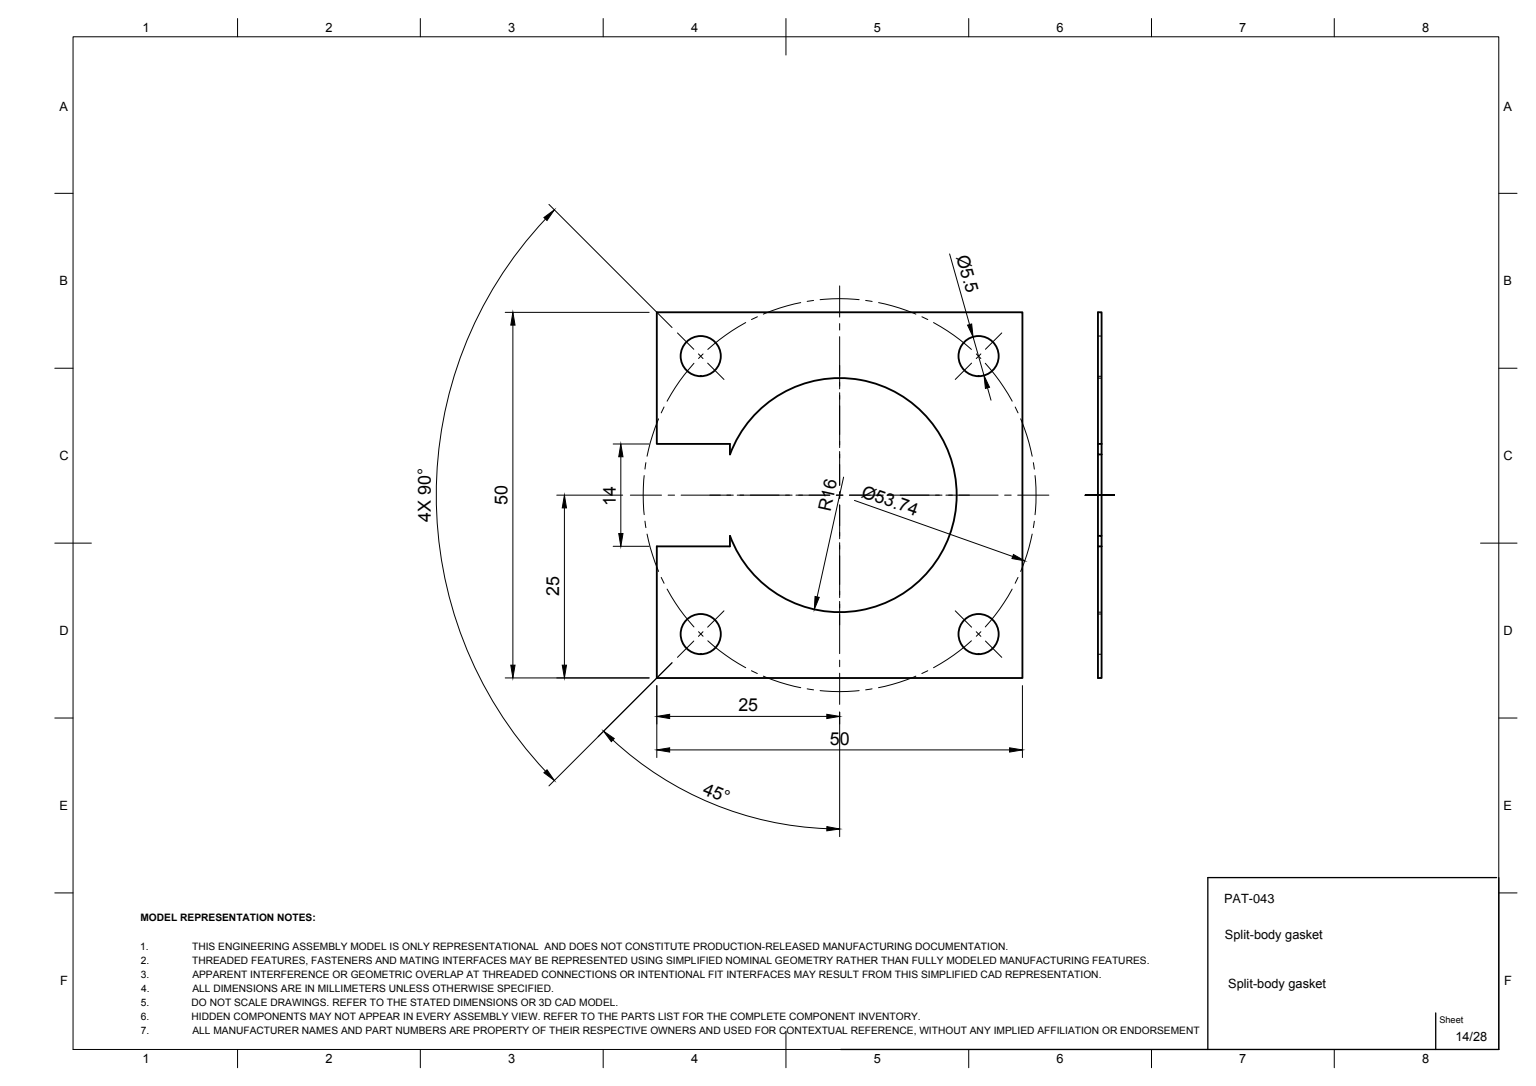
ISO-10303-21;
HEADER;
/* Generated by software containing ST-Developer
 * from STEP Tools, Inc. (www.steptools.com) 
 */

FILE_DESCRIPTION(
/* description */ ('Four-valve pipe header'),
/* implementation_level */ '2;1');

FILE_NAME(
/* name */ 'Split-body gasket.step',
/* time_stamp */ '2026-10-29T16:56:19-07:00',
/* author */ (''),
/* organization */ (''),
/* preprocessor_version */ 'ST-DEVELOPER v20.2',
/* originating_system */ 'Autodesk Translation Framework v15.17.0.0',
/* authorisation */ '');

FILE_SCHEMA (('AUTOMOTIVE_DESIGN { 1 0 10303 214 3 1 1 }'));
ENDSEC;

DATA;
#10=MECHANICAL_DESIGN_GEOMETRIC_PRESENTATION_REPRESENTATION('',(#340),#10119);
#288=SHAPE_REPRESENTATION_RELATIONSHIP('SRR','None',#10250,#314);
#314=ADVANCED_BREP_SHAPE_REPRESENTATION('',(#366),#10099);
#340=STYLED_ITEM('',(#10449),#366);
#366=MANIFOLD_SOLID_BREP('Body1',#5586);
#484=FACE_BOUND('',#1291,.T.);
#485=FACE_BOUND('',#1292,.T.);
#486=FACE_BOUND('',#1293,.T.);
#487=FACE_BOUND('',#1294,.T.);
#488=FACE_BOUND('',#1302,.T.);
#489=FACE_BOUND('',#1303,.T.);
#490=FACE_BOUND('',#1304,.T.);
#491=FACE_BOUND('',#1305,.T.);
#619=PLANE('',#6205);
#620=PLANE('',#6206);
#621=PLANE('',#6207);
#622=PLANE('',#6208);
#623=PLANE('',#6209);
#624=PLANE('',#6211);
#625=PLANE('',#6212);
#626=PLANE('',#6215);
#627=PLANE('',#6216);
#628=PLANE('',#6217);
#629=PLANE('',#6218);
#892=FACE_OUTER_BOUND('',#1282,.T.);
#893=FACE_OUTER_BOUND('',#1283,.T.);
#894=FACE_OUTER_BOUND('',#1284,.T.);
#895=FACE_OUTER_BOUND('',#1285,.T.);
#896=FACE_OUTER_BOUND('',#1286,.T.);
#897=FACE_OUTER_BOUND('',#1287,.T.);
#898=FACE_OUTER_BOUND('',#1288,.T.);
#899=FACE_OUTER_BOUND('',#1289,.T.);
#900=FACE_OUTER_BOUND('',#1290,.T.);
#901=FACE_OUTER_BOUND('',#1295,.T.);
#902=FACE_OUTER_BOUND('',#1296,.T.);
#903=FACE_OUTER_BOUND('',#1297,.T.);
#904=FACE_OUTER_BOUND('',#1298,.T.);
#905=FACE_OUTER_BOUND('',#1299,.T.);
#906=FACE_OUTER_BOUND('',#1300,.T.);
#907=FACE_OUTER_BOUND('',#1301,.T.);
#1282=EDGE_LOOP('',(#4399,#4400,#4401,#4402));
#1283=EDGE_LOOP('',(#4403,#4404,#4405,#4406));
#1284=EDGE_LOOP('',(#4407,#4408,#4409,#4410));
#1285=EDGE_LOOP('',(#4411,#4412,#4413,#4414));
#1286=EDGE_LOOP('',(#4415,#4416,#4417,#4418));
#1287=EDGE_LOOP('',(#4419,#4420,#4421,#4422));
#1288=EDGE_LOOP('',(#4423,#4424,#4425,#4426));
#1289=EDGE_LOOP('',(#4427,#4428,#4429,#4430));
#1290=EDGE_LOOP('',(#4431,#4432,#4433,#4434,#4435,#4436,#4437,#4438,#4439,
#4440));
#1291=EDGE_LOOP('',(#4441));
#1292=EDGE_LOOP('',(#4442));
#1293=EDGE_LOOP('',(#4443));
#1294=EDGE_LOOP('',(#4444));
#1295=EDGE_LOOP('',(#4445,#4446,#4447,#4448));
#1296=EDGE_LOOP('',(#4449,#4450,#4451,#4452));
#1297=EDGE_LOOP('',(#4453,#4454,#4455,#4456));
#1298=EDGE_LOOP('',(#4457,#4458,#4459,#4460));
#1299=EDGE_LOOP('',(#4461,#4462,#4463,#4464));
#1300=EDGE_LOOP('',(#4465,#4466,#4467,#4468));
#1301=EDGE_LOOP('',(#4469,#4470,#4471,#4472,#4473,#4474,#4475,#4476,#4477,
#4478));
#1302=EDGE_LOOP('',(#4479));
#1303=EDGE_LOOP('',(#4480));
#1304=EDGE_LOOP('',(#4481));
#1305=EDGE_LOOP('',(#4482));
#1689=LINE('',#9158,#2107);
#1690=LINE('',#9164,#2108);
#1691=LINE('',#9170,#2109);
#1692=LINE('',#9176,#2110);
#1693=LINE('',#9181,#2111);
#1694=LINE('',#9183,#2112);
#1695=LINE('',#9185,#2113);
#1696=LINE('',#9186,#2114);
#1697=LINE('',#9190,#2115);
#1698=LINE('',#9192,#2116);
#1699=LINE('',#9194,#2117);
#1700=LINE('',#9195,#2118);
#1701=LINE('',#9198,#2119);
#1702=LINE('',#9200,#2120);
#1703=LINE('',#9201,#2121);
#1704=LINE('',#9204,#2122);
#1705=LINE('',#9206,#2123);
#1706=LINE('',#9207,#2124);
#1707=LINE('',#9211,#2125);
#1708=LINE('',#9213,#2126);
#1709=LINE('',#9215,#2127);
#1710=LINE('',#9217,#2128);
#1711=LINE('',#9218,#2129);
#1712=LINE('',#9221,#2130);
#1713=LINE('',#9222,#2131);
#1714=LINE('',#9225,#2132);
#1715=LINE('',#9226,#2133);
#1716=LINE('',#9231,#2134);
#1717=LINE('',#9232,#2135);
#1718=LINE('',#9235,#2136);
#1719=LINE('',#9236,#2137);
#1720=LINE('',#9238,#2138);
#2107=VECTOR('',#7338,0.275);
#2108=VECTOR('',#7345,0.275);
#2109=VECTOR('',#7352,0.275);
#2110=VECTOR('',#7359,0.275);
#2111=VECTOR('',#7364,1.);
#2112=VECTOR('',#7365,1.);
#2113=VECTOR('',#7366,1.);
#2114=VECTOR('',#7367,1.);
#2115=VECTOR('',#7370,1.);
#2116=VECTOR('',#7371,1.);
#2117=VECTOR('',#7372,1.);
#2118=VECTOR('',#7373,1.);
#2119=VECTOR('',#7376,1.);
#2120=VECTOR('',#7377,1.);
#2121=VECTOR('',#7378,1.);
#2122=VECTOR('',#7381,1.);
#2123=VECTOR('',#7382,1.);
#2124=VECTOR('',#7383,1.);
#2125=VECTOR('',#7388,1.);
#2126=VECTOR('',#7389,1.);
#2127=VECTOR('',#7390,1.);
#2128=VECTOR('',#7391,1.);
#2129=VECTOR('',#7392,1.);
#2130=VECTOR('',#7395,1.);
#2131=VECTOR('',#7396,1.);
#2132=VECTOR('',#7399,1.);
#2133=VECTOR('',#7400,1.);
#2134=VECTOR('',#7407,1.);
#2135=VECTOR('',#7408,1.);
#2136=VECTOR('',#7411,1.);
#2137=VECTOR('',#7412,1.);
#2138=VECTOR('',#7415,1.);
#2466=CIRCLE('',#6194,0.275);
#2467=CIRCLE('',#6195,0.275);
#2468=CIRCLE('',#6197,0.275);
#2469=CIRCLE('',#6198,0.275);
#2470=CIRCLE('',#6200,0.275);
#2471=CIRCLE('',#6201,0.275);
#2472=CIRCLE('',#6203,0.275);
#2473=CIRCLE('',#6204,0.275);
#2474=CIRCLE('',#6210,1.6);
#2475=CIRCLE('',#6214,1.6);
#2794=VERTEX_POINT('',#9155);
#2795=VERTEX_POINT('',#9157);
#2796=VERTEX_POINT('',#9161);
#2797=VERTEX_POINT('',#9163);
#2798=VERTEX_POINT('',#9167);
#2799=VERTEX_POINT('',#9169);
#2800=VERTEX_POINT('',#9173);
#2801=VERTEX_POINT('',#9175);
#2802=VERTEX_POINT('',#9179);
#2803=VERTEX_POINT('',#9180);
#2804=VERTEX_POINT('',#9182);
#2805=VERTEX_POINT('',#9184);
#2806=VERTEX_POINT('',#9188);
#2807=VERTEX_POINT('',#9189);
#2808=VERTEX_POINT('',#9191);
#2809=VERTEX_POINT('',#9193);
#2810=VERTEX_POINT('',#9197);
#2811=VERTEX_POINT('',#9199);
#2812=VERTEX_POINT('',#9203);
#2813=VERTEX_POINT('',#9205);
#2814=VERTEX_POINT('',#9210);
#2815=VERTEX_POINT('',#9212);
#2816=VERTEX_POINT('',#9214);
#2817=VERTEX_POINT('',#9216);
#2818=VERTEX_POINT('',#9220);
#2819=VERTEX_POINT('',#9224);
#2820=VERTEX_POINT('',#9230);
#2821=VERTEX_POINT('',#9234);
#3366=EDGE_CURVE('',#2794,#2794,#2466,.T.);
#3367=EDGE_CURVE('',#2794,#2795,#1689,.T.);
#3368=EDGE_CURVE('',#2795,#2795,#2467,.T.);
#3369=EDGE_CURVE('',#2796,#2796,#2468,.T.);
#3370=EDGE_CURVE('',#2796,#2797,#1690,.T.);
#3371=EDGE_CURVE('',#2797,#2797,#2469,.T.);
#3372=EDGE_CURVE('',#2798,#2798,#2470,.T.);
#3373=EDGE_CURVE('',#2798,#2799,#1691,.T.);
#3374=EDGE_CURVE('',#2799,#2799,#2471,.T.);
#3375=EDGE_CURVE('',#2800,#2800,#2472,.T.);
#3376=EDGE_CURVE('',#2800,#2801,#1692,.T.);
#3377=EDGE_CURVE('',#2801,#2801,#2473,.T.);
#3378=EDGE_CURVE('',#2802,#2803,#1693,.T.);
#3379=EDGE_CURVE('',#2802,#2804,#1694,.T.);
#3380=EDGE_CURVE('',#2805,#2804,#1695,.T.);
#3381=EDGE_CURVE('',#2803,#2805,#1696,.T.);
#3382=EDGE_CURVE('',#2806,#2807,#1697,.T.);
#3383=EDGE_CURVE('',#2806,#2808,#1698,.T.);
#3384=EDGE_CURVE('',#2809,#2808,#1699,.T.);
#3385=EDGE_CURVE('',#2807,#2809,#1700,.T.);
#3386=EDGE_CURVE('',#2810,#2802,#1701,.T.);
#3387=EDGE_CURVE('',#2811,#2810,#1702,.T.);
#3388=EDGE_CURVE('',#2804,#2811,#1703,.T.);
#3389=EDGE_CURVE('',#2812,#2806,#1704,.T.);
#3390=EDGE_CURVE('',#2813,#2812,#1705,.T.);
#3391=EDGE_CURVE('',#2808,#2813,#1706,.T.);
#3392=EDGE_CURVE('',#2811,#2809,#2474,.T.);
#3393=EDGE_CURVE('',#2813,#2814,#1707,.T.);
#3394=EDGE_CURVE('',#2814,#2815,#1708,.T.);
#3395=EDGE_CURVE('',#2815,#2816,#1709,.T.);
#3396=EDGE_CURVE('',#2816,#2817,#1710,.T.);
#3397=EDGE_CURVE('',#2817,#2805,#1711,.T.);
#3398=EDGE_CURVE('',#2818,#2812,#1712,.T.);
#3399=EDGE_CURVE('',#2818,#2814,#1713,.T.);
#3400=EDGE_CURVE('',#2819,#2817,#1714,.T.);
#3401=EDGE_CURVE('',#2803,#2819,#1715,.T.);
#3402=EDGE_CURVE('',#2807,#2810,#2475,.T.);
#3403=EDGE_CURVE('',#2819,#2820,#1716,.T.);
#3404=EDGE_CURVE('',#2820,#2816,#1717,.T.);
#3405=EDGE_CURVE('',#2820,#2821,#1718,.T.);
#3406=EDGE_CURVE('',#2821,#2815,#1719,.T.);
#3407=EDGE_CURVE('',#2821,#2818,#1720,.T.);
#4399=ORIENTED_EDGE('',*,*,#3366,.F.);
#4400=ORIENTED_EDGE('',*,*,#3367,.T.);
#4401=ORIENTED_EDGE('',*,*,#3368,.F.);
#4402=ORIENTED_EDGE('',*,*,#3367,.F.);
#4403=ORIENTED_EDGE('',*,*,#3369,.F.);
#4404=ORIENTED_EDGE('',*,*,#3370,.T.);
#4405=ORIENTED_EDGE('',*,*,#3371,.F.);
#4406=ORIENTED_EDGE('',*,*,#3370,.F.);
#4407=ORIENTED_EDGE('',*,*,#3372,.F.);
#4408=ORIENTED_EDGE('',*,*,#3373,.T.);
#4409=ORIENTED_EDGE('',*,*,#3374,.F.);
#4410=ORIENTED_EDGE('',*,*,#3373,.F.);
#4411=ORIENTED_EDGE('',*,*,#3375,.F.);
#4412=ORIENTED_EDGE('',*,*,#3376,.T.);
#4413=ORIENTED_EDGE('',*,*,#3377,.F.);
#4414=ORIENTED_EDGE('',*,*,#3376,.F.);
#4415=ORIENTED_EDGE('',*,*,#3378,.F.);
#4416=ORIENTED_EDGE('',*,*,#3379,.T.);
#4417=ORIENTED_EDGE('',*,*,#3380,.F.);
#4418=ORIENTED_EDGE('',*,*,#3381,.F.);
#4419=ORIENTED_EDGE('',*,*,#3382,.F.);
#4420=ORIENTED_EDGE('',*,*,#3383,.T.);
#4421=ORIENTED_EDGE('',*,*,#3384,.F.);
#4422=ORIENTED_EDGE('',*,*,#3385,.F.);
#4423=ORIENTED_EDGE('',*,*,#3386,.F.);
#4424=ORIENTED_EDGE('',*,*,#3387,.F.);
#4425=ORIENTED_EDGE('',*,*,#3388,.F.);
#4426=ORIENTED_EDGE('',*,*,#3379,.F.);
#4427=ORIENTED_EDGE('',*,*,#3389,.F.);
#4428=ORIENTED_EDGE('',*,*,#3390,.F.);
#4429=ORIENTED_EDGE('',*,*,#3391,.F.);
#4430=ORIENTED_EDGE('',*,*,#3383,.F.);
#4431=ORIENTED_EDGE('',*,*,#3380,.T.);
#4432=ORIENTED_EDGE('',*,*,#3388,.T.);
#4433=ORIENTED_EDGE('',*,*,#3392,.T.);
#4434=ORIENTED_EDGE('',*,*,#3384,.T.);
#4435=ORIENTED_EDGE('',*,*,#3391,.T.);
#4436=ORIENTED_EDGE('',*,*,#3393,.T.);
#4437=ORIENTED_EDGE('',*,*,#3394,.T.);
#4438=ORIENTED_EDGE('',*,*,#3395,.T.);
#4439=ORIENTED_EDGE('',*,*,#3396,.T.);
#4440=ORIENTED_EDGE('',*,*,#3397,.T.);
#4441=ORIENTED_EDGE('',*,*,#3368,.T.);
#4442=ORIENTED_EDGE('',*,*,#3371,.T.);
#4443=ORIENTED_EDGE('',*,*,#3374,.T.);
#4444=ORIENTED_EDGE('',*,*,#3377,.T.);
#4445=ORIENTED_EDGE('',*,*,#3390,.T.);
#4446=ORIENTED_EDGE('',*,*,#3398,.F.);
#4447=ORIENTED_EDGE('',*,*,#3399,.T.);
#4448=ORIENTED_EDGE('',*,*,#3393,.F.);
#4449=ORIENTED_EDGE('',*,*,#3381,.T.);
#4450=ORIENTED_EDGE('',*,*,#3397,.F.);
#4451=ORIENTED_EDGE('',*,*,#3400,.F.);
#4452=ORIENTED_EDGE('',*,*,#3401,.F.);
#4453=ORIENTED_EDGE('',*,*,#3387,.T.);
#4454=ORIENTED_EDGE('',*,*,#3402,.F.);
#4455=ORIENTED_EDGE('',*,*,#3385,.T.);
#4456=ORIENTED_EDGE('',*,*,#3392,.F.);
#4457=ORIENTED_EDGE('',*,*,#3403,.F.);
#4458=ORIENTED_EDGE('',*,*,#3400,.T.);
#4459=ORIENTED_EDGE('',*,*,#3396,.F.);
#4460=ORIENTED_EDGE('',*,*,#3404,.F.);
#4461=ORIENTED_EDGE('',*,*,#3405,.F.);
#4462=ORIENTED_EDGE('',*,*,#3404,.T.);
#4463=ORIENTED_EDGE('',*,*,#3395,.F.);
#4464=ORIENTED_EDGE('',*,*,#3406,.F.);
#4465=ORIENTED_EDGE('',*,*,#3407,.F.);
#4466=ORIENTED_EDGE('',*,*,#3406,.T.);
#4467=ORIENTED_EDGE('',*,*,#3394,.F.);
#4468=ORIENTED_EDGE('',*,*,#3399,.F.);
#4469=ORIENTED_EDGE('',*,*,#3378,.T.);
#4470=ORIENTED_EDGE('',*,*,#3401,.T.);
#4471=ORIENTED_EDGE('',*,*,#3403,.T.);
#4472=ORIENTED_EDGE('',*,*,#3405,.T.);
#4473=ORIENTED_EDGE('',*,*,#3407,.T.);
#4474=ORIENTED_EDGE('',*,*,#3398,.T.);
#4475=ORIENTED_EDGE('',*,*,#3389,.T.);
#4476=ORIENTED_EDGE('',*,*,#3382,.T.);
#4477=ORIENTED_EDGE('',*,*,#3402,.T.);
#4478=ORIENTED_EDGE('',*,*,#3386,.T.);
#4479=ORIENTED_EDGE('',*,*,#3366,.T.);
#4480=ORIENTED_EDGE('',*,*,#3369,.T.);
#4481=ORIENTED_EDGE('',*,*,#3372,.T.);
#4482=ORIENTED_EDGE('',*,*,#3375,.T.);
#5206=CYLINDRICAL_SURFACE('',#6193,0.275);
#5207=CYLINDRICAL_SURFACE('',#6196,0.275);
#5208=CYLINDRICAL_SURFACE('',#6199,0.275);
#5209=CYLINDRICAL_SURFACE('',#6202,0.275);
#5210=CYLINDRICAL_SURFACE('',#6213,1.6);
#5392=ADVANCED_FACE('',(#892),#5206,.F.);
#5393=ADVANCED_FACE('',(#893),#5207,.F.);
#5394=ADVANCED_FACE('',(#894),#5208,.F.);
#5395=ADVANCED_FACE('',(#895),#5209,.F.);
#5396=ADVANCED_FACE('',(#896),#619,.F.);
#5397=ADVANCED_FACE('',(#897),#620,.F.);
#5398=ADVANCED_FACE('',(#898),#621,.F.);
#5399=ADVANCED_FACE('',(#899),#622,.F.);
#5400=ADVANCED_FACE('',(#900,#484,#485,#486,#487),#623,.T.);
#5401=ADVANCED_FACE('',(#901),#624,.T.);
#5402=ADVANCED_FACE('',(#902),#625,.T.);
#5403=ADVANCED_FACE('',(#903),#5210,.F.);
#5404=ADVANCED_FACE('',(#904),#626,.T.);
#5405=ADVANCED_FACE('',(#905),#627,.T.);
#5406=ADVANCED_FACE('',(#906),#628,.T.);
#5407=ADVANCED_FACE('',(#907,#488,#489,#490,#491),#629,.F.);
#5586=CLOSED_SHELL('',(#5392,#5393,#5394,#5395,#5396,#5397,#5398,#5399,
#5400,#5401,#5402,#5403,#5404,#5405,#5406,#5407));
#6192=AXIS2_PLACEMENT_3D('',#9153,#7332,#7333);
#6193=AXIS2_PLACEMENT_3D('',#9154,#7334,#7335);
#6194=AXIS2_PLACEMENT_3D('',#9156,#7336,#7337);
#6195=AXIS2_PLACEMENT_3D('',#9159,#7339,#7340);
#6196=AXIS2_PLACEMENT_3D('',#9160,#7341,#7342);
#6197=AXIS2_PLACEMENT_3D('',#9162,#7343,#7344);
#6198=AXIS2_PLACEMENT_3D('',#9165,#7346,#7347);
#6199=AXIS2_PLACEMENT_3D('',#9166,#7348,#7349);
#6200=AXIS2_PLACEMENT_3D('',#9168,#7350,#7351);
#6201=AXIS2_PLACEMENT_3D('',#9171,#7353,#7354);
#6202=AXIS2_PLACEMENT_3D('',#9172,#7355,#7356);
#6203=AXIS2_PLACEMENT_3D('',#9174,#7357,#7358);
#6204=AXIS2_PLACEMENT_3D('',#9177,#7360,#7361);
#6205=AXIS2_PLACEMENT_3D('',#9178,#7362,#7363);
#6206=AXIS2_PLACEMENT_3D('',#9187,#7368,#7369);
#6207=AXIS2_PLACEMENT_3D('',#9196,#7374,#7375);
#6208=AXIS2_PLACEMENT_3D('',#9202,#7379,#7380);
#6209=AXIS2_PLACEMENT_3D('',#9208,#7384,#7385);
#6210=AXIS2_PLACEMENT_3D('',#9209,#7386,#7387);
#6211=AXIS2_PLACEMENT_3D('',#9219,#7393,#7394);
#6212=AXIS2_PLACEMENT_3D('',#9223,#7397,#7398);
#6213=AXIS2_PLACEMENT_3D('',#9227,#7401,#7402);
#6214=AXIS2_PLACEMENT_3D('',#9228,#7403,#7404);
#6215=AXIS2_PLACEMENT_3D('',#9229,#7405,#7406);
#6216=AXIS2_PLACEMENT_3D('',#9233,#7409,#7410);
#6217=AXIS2_PLACEMENT_3D('',#9237,#7413,#7414);
#6218=AXIS2_PLACEMENT_3D('',#9239,#7416,#7417);
#7332=DIRECTION('axis',(0.,0.,1.));
#7333=DIRECTION('refdir',(1.,0.,0.));
#7334=DIRECTION('center_axis',(0.,1.,0.));
#7335=DIRECTION('ref_axis',(1.,0.,0.));
#7336=DIRECTION('center_axis',(0.,1.,0.));
#7337=DIRECTION('ref_axis',(1.,0.,0.));
#7338=DIRECTION('',(0.,1.,0.));
#7339=DIRECTION('center_axis',(0.,-1.,0.));
#7340=DIRECTION('ref_axis',(1.,0.,0.));
#7341=DIRECTION('center_axis',(0.,1.,0.));
#7342=DIRECTION('ref_axis',(1.,0.,0.));
#7343=DIRECTION('center_axis',(0.,1.,0.));
#7344=DIRECTION('ref_axis',(1.,0.,0.));
#7345=DIRECTION('',(0.,1.,0.));
#7346=DIRECTION('center_axis',(0.,-1.,0.));
#7347=DIRECTION('ref_axis',(1.,0.,0.));
#7348=DIRECTION('center_axis',(0.,1.,0.));
#7349=DIRECTION('ref_axis',(1.,0.,0.));
#7350=DIRECTION('center_axis',(0.,1.,0.));
#7351=DIRECTION('ref_axis',(1.,0.,0.));
#7352=DIRECTION('',(0.,1.,0.));
#7353=DIRECTION('center_axis',(0.,-1.,0.));
#7354=DIRECTION('ref_axis',(1.,0.,0.));
#7355=DIRECTION('center_axis',(0.,1.,0.));
#7356=DIRECTION('ref_axis',(1.,0.,0.));
#7357=DIRECTION('center_axis',(0.,1.,0.));
#7358=DIRECTION('ref_axis',(1.,0.,0.));
#7359=DIRECTION('',(0.,1.,0.));
#7360=DIRECTION('center_axis',(0.,-1.,0.));
#7361=DIRECTION('ref_axis',(1.,0.,0.));
#7362=DIRECTION('center_axis',(-1.,0.,0.));
#7363=DIRECTION('ref_axis',(0.,0.,1.));
#7364=DIRECTION('',(0.,0.,1.));
#7365=DIRECTION('',(0.,1.,0.));
#7366=DIRECTION('',(0.,0.,-1.));
#7367=DIRECTION('',(0.,1.,0.));
#7368=DIRECTION('center_axis',(0.,0.,-1.));
#7369=DIRECTION('ref_axis',(-1.,0.,0.));
#7370=DIRECTION('',(-1.,0.,0.));
#7371=DIRECTION('',(0.,1.,0.));
#7372=DIRECTION('',(1.,0.,0.));
#7373=DIRECTION('',(0.,1.,0.));
#7374=DIRECTION('center_axis',(0.,0.,-1.));
#7375=DIRECTION('ref_axis',(-1.,0.,0.));
#7376=DIRECTION('',(-1.,0.,0.));
#7377=DIRECTION('',(0.,-1.,0.));
#7378=DIRECTION('',(1.,0.,0.));
#7379=DIRECTION('center_axis',(1.,0.,0.));
#7380=DIRECTION('ref_axis',(0.,0.,-1.));
#7381=DIRECTION('',(0.,0.,-1.));
#7382=DIRECTION('',(0.,-1.,0.));
#7383=DIRECTION('',(0.,0.,1.));
#7384=DIRECTION('center_axis',(0.,1.,0.));
#7385=DIRECTION('ref_axis',(0.,0.,1.));
#7386=DIRECTION('center_axis',(0.,-1.,0.));
#7387=DIRECTION('ref_axis',(1.,0.,0.));
#7388=DIRECTION('',(1.,0.,0.));
#7389=DIRECTION('',(0.,0.,-1.));
#7390=DIRECTION('',(-1.,0.,0.));
#7391=DIRECTION('',(0.,0.,1.));
#7392=DIRECTION('',(1.,0.,0.));
#7393=DIRECTION('center_axis',(0.,0.,1.));
#7394=DIRECTION('ref_axis',(1.,0.,0.));
#7395=DIRECTION('',(-1.,0.,0.));
#7396=DIRECTION('',(0.,1.,0.));
#7397=DIRECTION('center_axis',(0.,0.,1.));
#7398=DIRECTION('ref_axis',(1.,0.,0.));
#7399=DIRECTION('',(0.,1.,0.));
#7400=DIRECTION('',(-1.,0.,0.));
#7401=DIRECTION('center_axis',(0.,1.,0.));
#7402=DIRECTION('ref_axis',(-1.83697019872103E-16,0.,-1.));
#7403=DIRECTION('center_axis',(0.,1.,0.));
#7404=DIRECTION('ref_axis',(1.,0.,0.));
#7405=DIRECTION('center_axis',(-1.,0.,0.));
#7406=DIRECTION('ref_axis',(0.,0.,1.));
#7407=DIRECTION('',(0.,0.,-1.));
#7408=DIRECTION('',(0.,1.,0.));
#7409=DIRECTION('center_axis',(0.,0.,-1.));
#7410=DIRECTION('ref_axis',(-1.,0.,0.));
#7411=DIRECTION('',(1.,0.,0.));
#7412=DIRECTION('',(0.,1.,0.));
#7413=DIRECTION('center_axis',(1.,0.,0.));
#7414=DIRECTION('ref_axis',(0.,0.,-1.));
#7415=DIRECTION('',(0.,0.,1.));
#7416=DIRECTION('center_axis',(0.,1.,0.));
#7417=DIRECTION('ref_axis',(1.,0.,0.));
#9153=CARTESIAN_POINT('',(0.,0.,0.));
#9154=CARTESIAN_POINT('Origin',(1.9,-0.1,3.1));
#9155=CARTESIAN_POINT('',(1.625,-0.025,3.1));
#9156=CARTESIAN_POINT('Origin',(1.9,-0.025,3.1));
#9157=CARTESIAN_POINT('',(1.625,0.025,3.1));
#9158=CARTESIAN_POINT('',(1.625,-0.1,3.1));
#9159=CARTESIAN_POINT('Origin',(1.9,0.025,3.1));
#9160=CARTESIAN_POINT('Origin',(-1.9,-0.1,6.9));
#9161=CARTESIAN_POINT('',(-2.175,-0.025,6.9));
#9162=CARTESIAN_POINT('Origin',(-1.9,-0.025,6.9));
#9163=CARTESIAN_POINT('',(-2.175,0.025,6.9));
#9164=CARTESIAN_POINT('',(-2.175,-0.1,6.9));
#9165=CARTESIAN_POINT('Origin',(-1.9,0.025,6.9));
#9166=CARTESIAN_POINT('Origin',(-1.9,-0.1,3.1));
#9167=CARTESIAN_POINT('',(-2.175,-0.025,3.1));
#9168=CARTESIAN_POINT('Origin',(-1.9,-0.025,3.1));
#9169=CARTESIAN_POINT('',(-2.175,0.025,3.1));
#9170=CARTESIAN_POINT('',(-2.175,-0.1,3.1));
#9171=CARTESIAN_POINT('Origin',(-1.9,0.025,3.1));
#9172=CARTESIAN_POINT('Origin',(1.9,-0.1,6.9));
#9173=CARTESIAN_POINT('',(1.625,-0.025,6.9));
#9174=CARTESIAN_POINT('Origin',(1.9,-0.025,6.9));
#9175=CARTESIAN_POINT('',(1.625,0.025,6.9));
#9176=CARTESIAN_POINT('',(1.625,-0.1,6.9));
#9177=CARTESIAN_POINT('Origin',(1.9,0.025,6.9));
#9178=CARTESIAN_POINT('Origin',(-0.7,-0.1,6.5));
#9179=CARTESIAN_POINT('',(-0.7,-0.025,6.5));
#9180=CARTESIAN_POINT('',(-0.7,-0.025,7.5));
#9181=CARTESIAN_POINT('',(-0.7,-0.025,5.75));
#9182=CARTESIAN_POINT('',(-0.7,0.025,6.5));
#9183=CARTESIAN_POINT('',(-0.7,-0.1,6.5));
#9184=CARTESIAN_POINT('',(-0.7,0.025,7.5));
#9185=CARTESIAN_POINT('',(-0.7,0.025,5.75));
#9186=CARTESIAN_POINT('',(-0.7,-0.0625,7.5));
#9187=CARTESIAN_POINT('Origin',(0.7,-0.1,6.5));
#9188=CARTESIAN_POINT('',(0.7,-0.025,6.5));
#9189=CARTESIAN_POINT('',(0.556776436283003,-0.025,6.5));
#9190=CARTESIAN_POINT('',(0.35,-0.025,6.5));
#9191=CARTESIAN_POINT('',(0.7,0.025,6.5));
#9192=CARTESIAN_POINT('',(0.7,-0.1,6.5));
#9193=CARTESIAN_POINT('',(0.556776436283003,0.025,6.5));
#9194=CARTESIAN_POINT('',(0.35,0.025,6.5));
#9195=CARTESIAN_POINT('',(0.556776436283003,-0.1,6.5));
#9196=CARTESIAN_POINT('Origin',(0.7,-0.1,6.5));
#9197=CARTESIAN_POINT('',(-0.556776436283003,-0.025,6.5));
#9198=CARTESIAN_POINT('',(0.35,-0.025,6.5));
#9199=CARTESIAN_POINT('',(-0.556776436283003,0.025,6.5));
#9200=CARTESIAN_POINT('',(-0.556776436283003,-0.1,6.5));
#9201=CARTESIAN_POINT('',(0.35,0.025,6.5));
#9202=CARTESIAN_POINT('Origin',(0.7,-0.1,7.6));
#9203=CARTESIAN_POINT('',(0.7,-0.025,7.5));
#9204=CARTESIAN_POINT('',(0.7,-0.025,6.3));
#9205=CARTESIAN_POINT('',(0.7,0.025,7.5));
#9206=CARTESIAN_POINT('',(0.7,-0.0625,7.5));
#9207=CARTESIAN_POINT('',(0.7,0.025,6.3));
#9208=CARTESIAN_POINT('Origin',(0.,0.025,5.));
#9209=CARTESIAN_POINT('Origin',(0.,0.025,5.));
#9210=CARTESIAN_POINT('',(2.5,0.025,7.5));
#9211=CARTESIAN_POINT('',(2.5,0.025,7.5));
#9212=CARTESIAN_POINT('',(2.5,0.025,2.5));
#9213=CARTESIAN_POINT('',(2.5,0.025,2.5));
#9214=CARTESIAN_POINT('',(-2.5,0.025,2.5));
#9215=CARTESIAN_POINT('',(-2.5,0.025,2.5));
#9216=CARTESIAN_POINT('',(-2.5,0.025,7.5));
#9217=CARTESIAN_POINT('',(-2.5,0.025,7.5));
#9218=CARTESIAN_POINT('',(2.5,0.025,7.5));
#9219=CARTESIAN_POINT('Origin',(-2.5,-0.025,7.5));
#9220=CARTESIAN_POINT('',(2.5,-0.025,7.5));
#9221=CARTESIAN_POINT('',(2.5,-0.025,7.5));
#9222=CARTESIAN_POINT('',(2.5,-0.025,7.5));
#9223=CARTESIAN_POINT('Origin',(-2.5,-0.025,7.5));
#9224=CARTESIAN_POINT('',(-2.5,-0.025,7.5));
#9225=CARTESIAN_POINT('',(-2.5,-0.025,7.5));
#9226=CARTESIAN_POINT('',(2.5,-0.025,7.5));
#9227=CARTESIAN_POINT('Origin',(0.,-0.1,5.));
#9228=CARTESIAN_POINT('Origin',(0.,-0.025,5.));
#9229=CARTESIAN_POINT('Origin',(-2.5,-0.025,2.5));
#9230=CARTESIAN_POINT('',(-2.5,-0.025,2.5));
#9231=CARTESIAN_POINT('',(-2.5,-0.025,7.5));
#9232=CARTESIAN_POINT('',(-2.5,-0.025,2.5));
#9233=CARTESIAN_POINT('Origin',(2.5,-0.025,2.5));
#9234=CARTESIAN_POINT('',(2.5,-0.025,2.5));
#9235=CARTESIAN_POINT('',(-2.5,-0.025,2.5));
#9236=CARTESIAN_POINT('',(2.5,-0.025,2.5));
#9237=CARTESIAN_POINT('Origin',(2.5,-0.025,7.5));
#9238=CARTESIAN_POINT('',(2.5,-0.025,2.5));
#9239=CARTESIAN_POINT('Origin',(0.,-0.025,5.));
#10068=UNCERTAINTY_MEASURE_WITH_UNIT(LENGTH_MEASURE(0.001),#10120,
'DISTANCE_ACCURACY_VALUE',
'Maximum model space distance between geometric entities at asserted c
onnectivities');
#10088=UNCERTAINTY_MEASURE_WITH_UNIT(LENGTH_MEASURE(0.001),#10120,
'DISTANCE_ACCURACY_VALUE',
'Maximum model space distance between geometric entities at asserted c
onnectivities');
#10099=(
GEOMETRIC_REPRESENTATION_CONTEXT(3)
GLOBAL_UNCERTAINTY_ASSIGNED_CONTEXT((#10068))
GLOBAL_UNIT_ASSIGNED_CONTEXT((#10120,#10122,#10123))
REPRESENTATION_CONTEXT('','3D')
);
#10119=(
GEOMETRIC_REPRESENTATION_CONTEXT(3)
GLOBAL_UNCERTAINTY_ASSIGNED_CONTEXT((#10088))
GLOBAL_UNIT_ASSIGNED_CONTEXT((#10120,#10122,#10123))
REPRESENTATION_CONTEXT('','3D')
);
#10120=(
LENGTH_UNIT()
NAMED_UNIT(*)
SI_UNIT(.CENTI.,.METRE.)
);
#10122=(
NAMED_UNIT(*)
PLANE_ANGLE_UNIT()
SI_UNIT($,.RADIAN.)
);
#10123=(
NAMED_UNIT(*)
SI_UNIT($,.STERADIAN.)
SOLID_ANGLE_UNIT()
);
#10134=SHAPE_DEFINITION_REPRESENTATION(#10164,#10250);
#10164=PRODUCT_DEFINITION_SHAPE('',$,#10281);
#10250=SHAPE_REPRESENTATION('',(#6192),#10099);
#10270=PRODUCT_DEFINITION_CONTEXT('part definition',#10362,'design');
#10281=PRODUCT_DEFINITION('Split-body gasket','Split-body gasket',#10311,
#10270);
#10311=PRODUCT_DEFINITION_FORMATION('',$,#10374);
#10362=APPLICATION_CONTEXT(
'Core Data for Automotive Mechanical Design Process');
#10363=PRODUCT_CONTEXT('part definition',#10362,'mechanical');
#10374=PRODUCT('Split-body gasket','Split-body gasket',
'Split-body gasket',(#10363));
#10443=COLOUR_RGB('Dark Blue',0.08,0.2,0.34);
#10444=FILL_AREA_STYLE_COLOUR('',#10443);
#10445=FILL_AREA_STYLE('',(#10444));
#10446=SURFACE_STYLE_FILL_AREA(#10445);
#10447=SURFACE_SIDE_STYLE('',(#10446));
#10448=SURFACE_STYLE_USAGE(.BOTH.,#10447);
#10449=PRESENTATION_STYLE_ASSIGNMENT((#10448));
ENDSEC;
END-ISO-10303-21;
